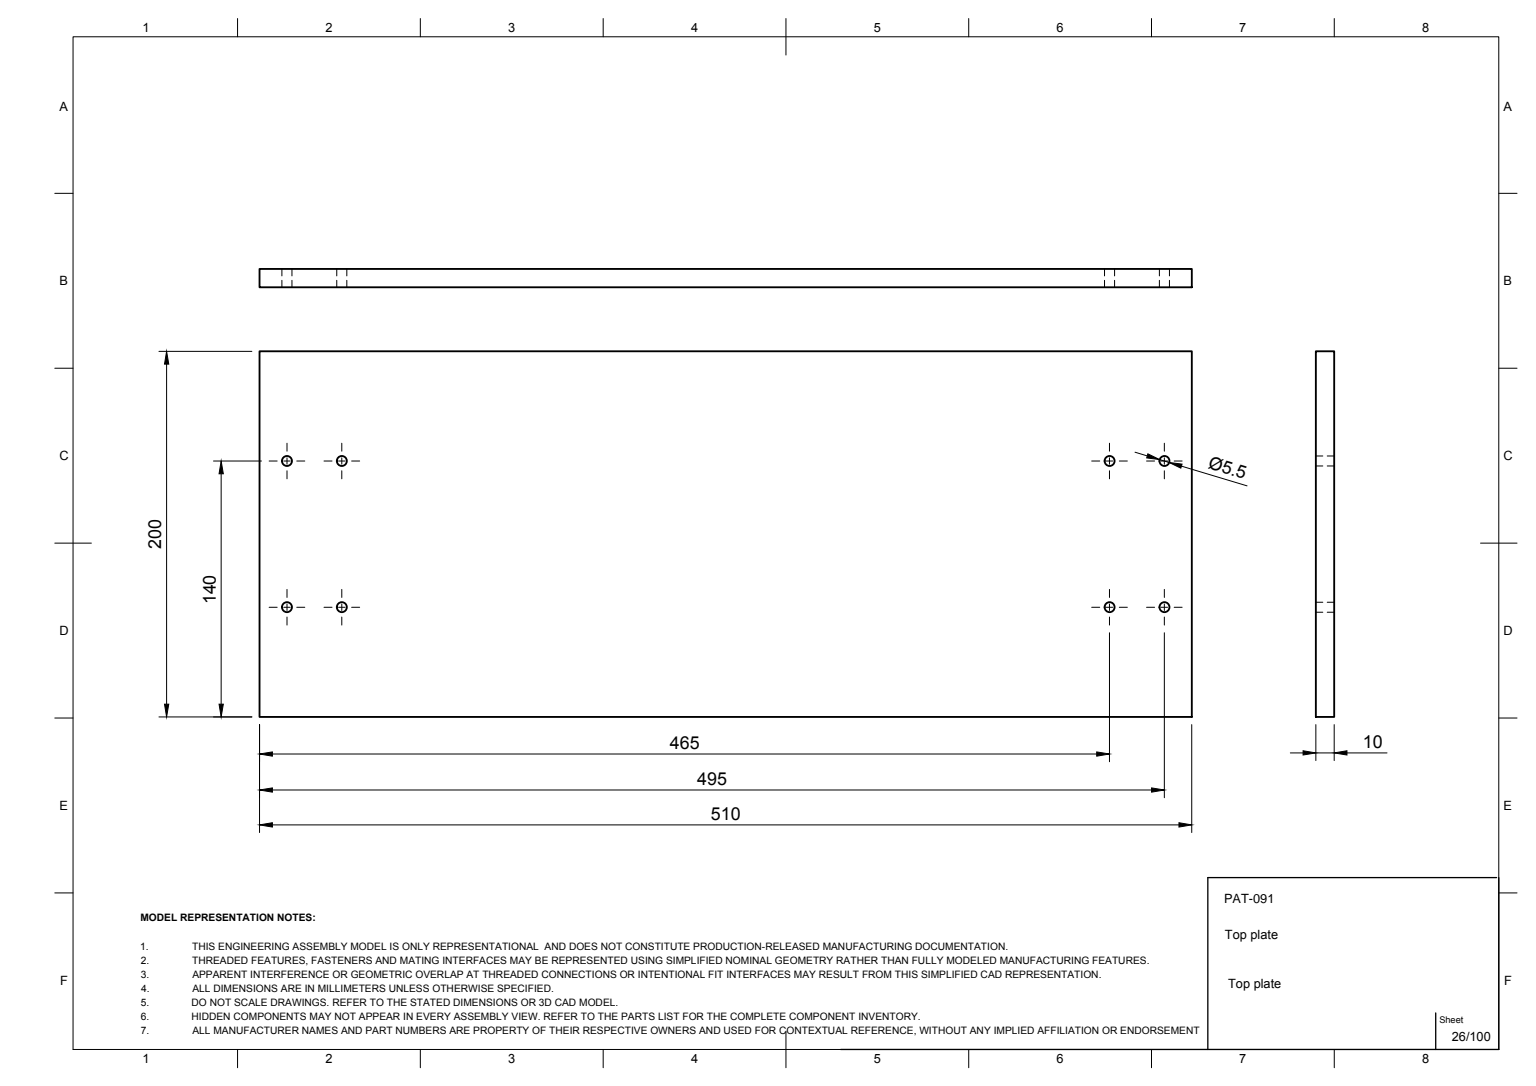
ISO-10303-21;
HEADER;
/* Generated by software containing ST-Developer
 * from STEP Tools, Inc. (www.steptools.com) 
 */

FILE_DESCRIPTION(
/* description */ ('PAT-091'),
/* implementation_level */ '2;1');

FILE_NAME(
/* name */ 'Top plate.step',
/* time_stamp */ '2026-10-27T15:34:44-07:00',
/* author */ (''),
/* organization */ (''),
/* preprocessor_version */ 'ST-DEVELOPER v20.2',
/* originating_system */ 'Autodesk Translation Framework v15.17.0.0',
/* authorisation */ '');

FILE_SCHEMA (('AUTOMOTIVE_DESIGN { 1 0 10303 214 3 1 1 }'));
ENDSEC;

DATA;
#10=MECHANICAL_DESIGN_GEOMETRIC_PRESENTATION_REPRESENTATION('',(#989),#25100);
#769=SHAPE_REPRESENTATION_RELATIONSHIP('SRR','None',#25531,#879);
#879=ADVANCED_BREP_SHAPE_REPRESENTATION('',(#1112),#25001);
#989=STYLED_ITEM('',(#26177),#1112);
#1112=MANIFOLD_SOLID_BREP('Body1',#13267);
#1334=FACE_BOUND('',#3171,.T.);
#1335=FACE_BOUND('',#3172,.T.);
#1336=FACE_BOUND('',#3173,.T.);
#1337=FACE_BOUND('',#3174,.T.);
#1338=FACE_BOUND('',#3175,.T.);
#1339=FACE_BOUND('',#3176,.T.);
#1340=FACE_BOUND('',#3177,.T.);
#1341=FACE_BOUND('',#3178,.T.);
#1342=FACE_BOUND('',#3180,.T.);
#1343=FACE_BOUND('',#3181,.T.);
#1344=FACE_BOUND('',#3182,.T.);
#1345=FACE_BOUND('',#3183,.T.);
#1346=FACE_BOUND('',#3184,.T.);
#1347=FACE_BOUND('',#3185,.T.);
#1348=FACE_BOUND('',#3186,.T.);
#1349=FACE_BOUND('',#3187,.T.);
#1719=PLANE('',#14944);
#1720=PLANE('',#14945);
#1721=PLANE('',#14946);
#1722=PLANE('',#14947);
#1723=PLANE('',#14948);
#1724=PLANE('',#14949);
#2221=FACE_OUTER_BOUND('',#3158,.T.);
#2222=FACE_OUTER_BOUND('',#3159,.T.);
#2223=FACE_OUTER_BOUND('',#3160,.T.);
#2224=FACE_OUTER_BOUND('',#3161,.T.);
#2225=FACE_OUTER_BOUND('',#3162,.T.);
#2226=FACE_OUTER_BOUND('',#3163,.T.);
#2227=FACE_OUTER_BOUND('',#3164,.T.);
#2228=FACE_OUTER_BOUND('',#3165,.T.);
#2229=FACE_OUTER_BOUND('',#3166,.T.);
#2230=FACE_OUTER_BOUND('',#3167,.T.);
#2231=FACE_OUTER_BOUND('',#3168,.T.);
#2232=FACE_OUTER_BOUND('',#3169,.T.);
#2233=FACE_OUTER_BOUND('',#3170,.T.);
#2234=FACE_OUTER_BOUND('',#3179,.T.);
#3158=EDGE_LOOP('',(#9644,#9645,#9646,#9647));
#3159=EDGE_LOOP('',(#9648,#9649,#9650,#9651));
#3160=EDGE_LOOP('',(#9652,#9653,#9654,#9655));
#3161=EDGE_LOOP('',(#9656,#9657,#9658,#9659));
#3162=EDGE_LOOP('',(#9660,#9661,#9662,#9663));
#3163=EDGE_LOOP('',(#9664,#9665,#9666,#9667));
#3164=EDGE_LOOP('',(#9668,#9669,#9670,#9671));
#3165=EDGE_LOOP('',(#9672,#9673,#9674,#9675));
#3166=EDGE_LOOP('',(#9676,#9677,#9678,#9679));
#3167=EDGE_LOOP('',(#9680,#9681,#9682,#9683));
#3168=EDGE_LOOP('',(#9684,#9685,#9686,#9687));
#3169=EDGE_LOOP('',(#9688,#9689,#9690,#9691));
#3170=EDGE_LOOP('',(#9692,#9693,#9694,#9695));
#3171=EDGE_LOOP('',(#9696));
#3172=EDGE_LOOP('',(#9697));
#3173=EDGE_LOOP('',(#9698));
#3174=EDGE_LOOP('',(#9699));
#3175=EDGE_LOOP('',(#9700));
#3176=EDGE_LOOP('',(#9701));
#3177=EDGE_LOOP('',(#9702));
#3178=EDGE_LOOP('',(#9703));
#3179=EDGE_LOOP('',(#9704,#9705,#9706,#9707));
#3180=EDGE_LOOP('',(#9708));
#3181=EDGE_LOOP('',(#9709));
#3182=EDGE_LOOP('',(#9710));
#3183=EDGE_LOOP('',(#9711));
#3184=EDGE_LOOP('',(#9712));
#3185=EDGE_LOOP('',(#9713));
#3186=EDGE_LOOP('',(#9714));
#3187=EDGE_LOOP('',(#9715));
#4305=LINE('',#21717,#5045);
#4306=LINE('',#21723,#5046);
#4307=LINE('',#21729,#5047);
#4308=LINE('',#21735,#5048);
#4309=LINE('',#21741,#5049);
#4310=LINE('',#21747,#5050);
#4311=LINE('',#21753,#5051);
#4312=LINE('',#21759,#5052);
#4313=LINE('',#21764,#5053);
#4314=LINE('',#21766,#5054);
#4315=LINE('',#21768,#5055);
#4316=LINE('',#21769,#5056);
#4317=LINE('',#21772,#5057);
#4318=LINE('',#21774,#5058);
#4319=LINE('',#21775,#5059);
#4320=LINE('',#21778,#5060);
#4321=LINE('',#21780,#5061);
#4322=LINE('',#21781,#5062);
#4323=LINE('',#21783,#5063);
#4324=LINE('',#21784,#5064);
#5045=VECTOR('',#17323,0.274999999999999);
#5046=VECTOR('',#17330,0.274999999999999);
#5047=VECTOR('',#17337,0.274999999999999);
#5048=VECTOR('',#17344,0.274999999999999);
#5049=VECTOR('',#17351,0.275);
#5050=VECTOR('',#17358,0.275);
#5051=VECTOR('',#17365,0.275);
#5052=VECTOR('',#17372,0.275);
#5053=VECTOR('',#17377,1.);
#5054=VECTOR('',#17378,1.);
#5055=VECTOR('',#17379,1.);
#5056=VECTOR('',#17380,1.);
#5057=VECTOR('',#17383,1.);
#5058=VECTOR('',#17384,1.);
#5059=VECTOR('',#17385,1.);
#5060=VECTOR('',#17388,1.);
#5061=VECTOR('',#17389,1.);
#5062=VECTOR('',#17390,1.);
#5063=VECTOR('',#17393,1.);
#5064=VECTOR('',#17394,1.);
#5759=CIRCLE('',#14921,0.274999999999999);
#5760=CIRCLE('',#14922,0.274999999999999);
#5761=CIRCLE('',#14924,0.274999999999999);
#5762=CIRCLE('',#14925,0.274999999999999);
#5763=CIRCLE('',#14927,0.274999999999999);
#5764=CIRCLE('',#14928,0.274999999999999);
#5765=CIRCLE('',#14930,0.274999999999999);
#5766=CIRCLE('',#14931,0.274999999999999);
#5767=CIRCLE('',#14933,0.275);
#5768=CIRCLE('',#14934,0.275);
#5769=CIRCLE('',#14936,0.275);
#5770=CIRCLE('',#14937,0.275);
#5771=CIRCLE('',#14939,0.275);
#5772=CIRCLE('',#14940,0.275);
#5773=CIRCLE('',#14942,0.275);
#5774=CIRCLE('',#14943,0.275);
#6606=VERTEX_POINT('',#21714);
#6607=VERTEX_POINT('',#21716);
#6608=VERTEX_POINT('',#21720);
#6609=VERTEX_POINT('',#21722);
#6610=VERTEX_POINT('',#21726);
#6611=VERTEX_POINT('',#21728);
#6612=VERTEX_POINT('',#21732);
#6613=VERTEX_POINT('',#21734);
#6614=VERTEX_POINT('',#21738);
#6615=VERTEX_POINT('',#21740);
#6616=VERTEX_POINT('',#21744);
#6617=VERTEX_POINT('',#21746);
#6618=VERTEX_POINT('',#21750);
#6619=VERTEX_POINT('',#21752);
#6620=VERTEX_POINT('',#21756);
#6621=VERTEX_POINT('',#21758);
#6622=VERTEX_POINT('',#21762);
#6623=VERTEX_POINT('',#21763);
#6624=VERTEX_POINT('',#21765);
#6625=VERTEX_POINT('',#21767);
#6626=VERTEX_POINT('',#21771);
#6627=VERTEX_POINT('',#21773);
#6628=VERTEX_POINT('',#21777);
#6629=VERTEX_POINT('',#21779);
#7757=EDGE_CURVE('',#6606,#6606,#5759,.T.);
#7758=EDGE_CURVE('',#6606,#6607,#4305,.T.);
#7759=EDGE_CURVE('',#6607,#6607,#5760,.T.);
#7760=EDGE_CURVE('',#6608,#6608,#5761,.T.);
#7761=EDGE_CURVE('',#6608,#6609,#4306,.T.);
#7762=EDGE_CURVE('',#6609,#6609,#5762,.T.);
#7763=EDGE_CURVE('',#6610,#6610,#5763,.T.);
#7764=EDGE_CURVE('',#6610,#6611,#4307,.T.);
#7765=EDGE_CURVE('',#6611,#6611,#5764,.T.);
#7766=EDGE_CURVE('',#6612,#6612,#5765,.T.);
#7767=EDGE_CURVE('',#6612,#6613,#4308,.T.);
#7768=EDGE_CURVE('',#6613,#6613,#5766,.T.);
#7769=EDGE_CURVE('',#6614,#6614,#5767,.T.);
#7770=EDGE_CURVE('',#6614,#6615,#4309,.T.);
#7771=EDGE_CURVE('',#6615,#6615,#5768,.T.);
#7772=EDGE_CURVE('',#6616,#6616,#5769,.T.);
#7773=EDGE_CURVE('',#6616,#6617,#4310,.T.);
#7774=EDGE_CURVE('',#6617,#6617,#5770,.T.);
#7775=EDGE_CURVE('',#6618,#6618,#5771,.T.);
#7776=EDGE_CURVE('',#6618,#6619,#4311,.T.);
#7777=EDGE_CURVE('',#6619,#6619,#5772,.T.);
#7778=EDGE_CURVE('',#6620,#6620,#5773,.T.);
#7779=EDGE_CURVE('',#6620,#6621,#4312,.T.);
#7780=EDGE_CURVE('',#6621,#6621,#5774,.T.);
#7781=EDGE_CURVE('',#6622,#6623,#4313,.T.);
#7782=EDGE_CURVE('',#6623,#6624,#4314,.T.);
#7783=EDGE_CURVE('',#6625,#6624,#4315,.T.);
#7784=EDGE_CURVE('',#6622,#6625,#4316,.T.);
#7785=EDGE_CURVE('',#6626,#6622,#4317,.T.);
#7786=EDGE_CURVE('',#6627,#6625,#4318,.T.);
#7787=EDGE_CURVE('',#6626,#6627,#4319,.T.);
#7788=EDGE_CURVE('',#6628,#6626,#4320,.T.);
#7789=EDGE_CURVE('',#6629,#6627,#4321,.T.);
#7790=EDGE_CURVE('',#6628,#6629,#4322,.T.);
#7791=EDGE_CURVE('',#6623,#6628,#4323,.T.);
#7792=EDGE_CURVE('',#6624,#6629,#4324,.T.);
#9644=ORIENTED_EDGE('',*,*,#7757,.F.);
#9645=ORIENTED_EDGE('',*,*,#7758,.T.);
#9646=ORIENTED_EDGE('',*,*,#7759,.F.);
#9647=ORIENTED_EDGE('',*,*,#7758,.F.);
#9648=ORIENTED_EDGE('',*,*,#7760,.F.);
#9649=ORIENTED_EDGE('',*,*,#7761,.T.);
#9650=ORIENTED_EDGE('',*,*,#7762,.F.);
#9651=ORIENTED_EDGE('',*,*,#7761,.F.);
#9652=ORIENTED_EDGE('',*,*,#7763,.F.);
#9653=ORIENTED_EDGE('',*,*,#7764,.T.);
#9654=ORIENTED_EDGE('',*,*,#7765,.F.);
#9655=ORIENTED_EDGE('',*,*,#7764,.F.);
#9656=ORIENTED_EDGE('',*,*,#7766,.F.);
#9657=ORIENTED_EDGE('',*,*,#7767,.T.);
#9658=ORIENTED_EDGE('',*,*,#7768,.F.);
#9659=ORIENTED_EDGE('',*,*,#7767,.F.);
#9660=ORIENTED_EDGE('',*,*,#7769,.F.);
#9661=ORIENTED_EDGE('',*,*,#7770,.T.);
#9662=ORIENTED_EDGE('',*,*,#7771,.F.);
#9663=ORIENTED_EDGE('',*,*,#7770,.F.);
#9664=ORIENTED_EDGE('',*,*,#7772,.F.);
#9665=ORIENTED_EDGE('',*,*,#7773,.T.);
#9666=ORIENTED_EDGE('',*,*,#7774,.F.);
#9667=ORIENTED_EDGE('',*,*,#7773,.F.);
#9668=ORIENTED_EDGE('',*,*,#7775,.F.);
#9669=ORIENTED_EDGE('',*,*,#7776,.T.);
#9670=ORIENTED_EDGE('',*,*,#7777,.F.);
#9671=ORIENTED_EDGE('',*,*,#7776,.F.);
#9672=ORIENTED_EDGE('',*,*,#7778,.F.);
#9673=ORIENTED_EDGE('',*,*,#7779,.T.);
#9674=ORIENTED_EDGE('',*,*,#7780,.F.);
#9675=ORIENTED_EDGE('',*,*,#7779,.F.);
#9676=ORIENTED_EDGE('',*,*,#7781,.T.);
#9677=ORIENTED_EDGE('',*,*,#7782,.T.);
#9678=ORIENTED_EDGE('',*,*,#7783,.F.);
#9679=ORIENTED_EDGE('',*,*,#7784,.F.);
#9680=ORIENTED_EDGE('',*,*,#7785,.T.);
#9681=ORIENTED_EDGE('',*,*,#7784,.T.);
#9682=ORIENTED_EDGE('',*,*,#7786,.F.);
#9683=ORIENTED_EDGE('',*,*,#7787,.F.);
#9684=ORIENTED_EDGE('',*,*,#7788,.T.);
#9685=ORIENTED_EDGE('',*,*,#7787,.T.);
#9686=ORIENTED_EDGE('',*,*,#7789,.F.);
#9687=ORIENTED_EDGE('',*,*,#7790,.F.);
#9688=ORIENTED_EDGE('',*,*,#7791,.T.);
#9689=ORIENTED_EDGE('',*,*,#7790,.T.);
#9690=ORIENTED_EDGE('',*,*,#7792,.F.);
#9691=ORIENTED_EDGE('',*,*,#7782,.F.);
#9692=ORIENTED_EDGE('',*,*,#7792,.T.);
#9693=ORIENTED_EDGE('',*,*,#7789,.T.);
#9694=ORIENTED_EDGE('',*,*,#7786,.T.);
#9695=ORIENTED_EDGE('',*,*,#7783,.T.);
#9696=ORIENTED_EDGE('',*,*,#7780,.T.);
#9697=ORIENTED_EDGE('',*,*,#7777,.T.);
#9698=ORIENTED_EDGE('',*,*,#7774,.T.);
#9699=ORIENTED_EDGE('',*,*,#7771,.T.);
#9700=ORIENTED_EDGE('',*,*,#7768,.T.);
#9701=ORIENTED_EDGE('',*,*,#7765,.T.);
#9702=ORIENTED_EDGE('',*,*,#7762,.T.);
#9703=ORIENTED_EDGE('',*,*,#7759,.T.);
#9704=ORIENTED_EDGE('',*,*,#7791,.F.);
#9705=ORIENTED_EDGE('',*,*,#7781,.F.);
#9706=ORIENTED_EDGE('',*,*,#7785,.F.);
#9707=ORIENTED_EDGE('',*,*,#7788,.F.);
#9708=ORIENTED_EDGE('',*,*,#7778,.T.);
#9709=ORIENTED_EDGE('',*,*,#7775,.T.);
#9710=ORIENTED_EDGE('',*,*,#7772,.T.);
#9711=ORIENTED_EDGE('',*,*,#7769,.T.);
#9712=ORIENTED_EDGE('',*,*,#7766,.T.);
#9713=ORIENTED_EDGE('',*,*,#7763,.T.);
#9714=ORIENTED_EDGE('',*,*,#7760,.T.);
#9715=ORIENTED_EDGE('',*,*,#7757,.T.);
#12150=CYLINDRICAL_SURFACE('',#14920,0.274999999999999);
#12151=CYLINDRICAL_SURFACE('',#14923,0.274999999999999);
#12152=CYLINDRICAL_SURFACE('',#14926,0.274999999999999);
#12153=CYLINDRICAL_SURFACE('',#14929,0.274999999999999);
#12154=CYLINDRICAL_SURFACE('',#14932,0.275);
#12155=CYLINDRICAL_SURFACE('',#14935,0.275);
#12156=CYLINDRICAL_SURFACE('',#14938,0.275);
#12157=CYLINDRICAL_SURFACE('',#14941,0.275);
#12588=ADVANCED_FACE('',(#2221),#12150,.F.);
#12589=ADVANCED_FACE('',(#2222),#12151,.F.);
#12590=ADVANCED_FACE('',(#2223),#12152,.F.);
#12591=ADVANCED_FACE('',(#2224),#12153,.F.);
#12592=ADVANCED_FACE('',(#2225),#12154,.F.);
#12593=ADVANCED_FACE('',(#2226),#12155,.F.);
#12594=ADVANCED_FACE('',(#2227),#12156,.F.);
#12595=ADVANCED_FACE('',(#2228),#12157,.F.);
#12596=ADVANCED_FACE('',(#2229),#1719,.T.);
#12597=ADVANCED_FACE('',(#2230),#1720,.T.);
#12598=ADVANCED_FACE('',(#2231),#1721,.T.);
#12599=ADVANCED_FACE('',(#2232),#1722,.T.);
#12600=ADVANCED_FACE('',(#2233,#1334,#1335,#1336,#1337,#1338,#1339,#1340,
#1341),#1723,.T.);
#12601=ADVANCED_FACE('',(#2234,#1342,#1343,#1344,#1345,#1346,#1347,#1348,
#1349),#1724,.F.);
#13267=CLOSED_SHELL('',(#12588,#12589,#12590,#12591,#12592,#12593,#12594,
#12595,#12596,#12597,#12598,#12599,#12600,#12601));
#14919=AXIS2_PLACEMENT_3D('',#21712,#17317,#17318);
#14920=AXIS2_PLACEMENT_3D('',#21713,#17319,#17320);
#14921=AXIS2_PLACEMENT_3D('',#21715,#17321,#17322);
#14922=AXIS2_PLACEMENT_3D('',#21718,#17324,#17325);
#14923=AXIS2_PLACEMENT_3D('',#21719,#17326,#17327);
#14924=AXIS2_PLACEMENT_3D('',#21721,#17328,#17329);
#14925=AXIS2_PLACEMENT_3D('',#21724,#17331,#17332);
#14926=AXIS2_PLACEMENT_3D('',#21725,#17333,#17334);
#14927=AXIS2_PLACEMENT_3D('',#21727,#17335,#17336);
#14928=AXIS2_PLACEMENT_3D('',#21730,#17338,#17339);
#14929=AXIS2_PLACEMENT_3D('',#21731,#17340,#17341);
#14930=AXIS2_PLACEMENT_3D('',#21733,#17342,#17343);
#14931=AXIS2_PLACEMENT_3D('',#21736,#17345,#17346);
#14932=AXIS2_PLACEMENT_3D('',#21737,#17347,#17348);
#14933=AXIS2_PLACEMENT_3D('',#21739,#17349,#17350);
#14934=AXIS2_PLACEMENT_3D('',#21742,#17352,#17353);
#14935=AXIS2_PLACEMENT_3D('',#21743,#17354,#17355);
#14936=AXIS2_PLACEMENT_3D('',#21745,#17356,#17357);
#14937=AXIS2_PLACEMENT_3D('',#21748,#17359,#17360);
#14938=AXIS2_PLACEMENT_3D('',#21749,#17361,#17362);
#14939=AXIS2_PLACEMENT_3D('',#21751,#17363,#17364);
#14940=AXIS2_PLACEMENT_3D('',#21754,#17366,#17367);
#14941=AXIS2_PLACEMENT_3D('',#21755,#17368,#17369);
#14942=AXIS2_PLACEMENT_3D('',#21757,#17370,#17371);
#14943=AXIS2_PLACEMENT_3D('',#21760,#17373,#17374);
#14944=AXIS2_PLACEMENT_3D('',#21761,#17375,#17376);
#14945=AXIS2_PLACEMENT_3D('',#21770,#17381,#17382);
#14946=AXIS2_PLACEMENT_3D('',#21776,#17386,#17387);
#14947=AXIS2_PLACEMENT_3D('',#21782,#17391,#17392);
#14948=AXIS2_PLACEMENT_3D('',#21785,#17395,#17396);
#14949=AXIS2_PLACEMENT_3D('',#21786,#17397,#17398);
#17317=DIRECTION('axis',(0.,0.,1.));
#17318=DIRECTION('refdir',(1.,0.,0.));
#17319=DIRECTION('center_axis',(0.,0.,1.));
#17320=DIRECTION('ref_axis',(1.,0.,0.));
#17321=DIRECTION('center_axis',(0.,0.,1.));
#17322=DIRECTION('ref_axis',(1.,0.,0.));
#17323=DIRECTION('',(0.,0.,1.));
#17324=DIRECTION('center_axis',(0.,0.,-1.));
#17325=DIRECTION('ref_axis',(1.,0.,0.));
#17326=DIRECTION('center_axis',(0.,0.,1.));
#17327=DIRECTION('ref_axis',(1.,0.,0.));
#17328=DIRECTION('center_axis',(0.,0.,1.));
#17329=DIRECTION('ref_axis',(1.,0.,0.));
#17330=DIRECTION('',(0.,0.,1.));
#17331=DIRECTION('center_axis',(0.,0.,-1.));
#17332=DIRECTION('ref_axis',(1.,0.,0.));
#17333=DIRECTION('center_axis',(0.,0.,1.));
#17334=DIRECTION('ref_axis',(1.,0.,0.));
#17335=DIRECTION('center_axis',(0.,0.,1.));
#17336=DIRECTION('ref_axis',(1.,0.,0.));
#17337=DIRECTION('',(0.,0.,1.));
#17338=DIRECTION('center_axis',(0.,0.,-1.));
#17339=DIRECTION('ref_axis',(1.,0.,0.));
#17340=DIRECTION('center_axis',(0.,0.,1.));
#17341=DIRECTION('ref_axis',(1.,0.,0.));
#17342=DIRECTION('center_axis',(0.,0.,1.));
#17343=DIRECTION('ref_axis',(1.,0.,0.));
#17344=DIRECTION('',(0.,0.,1.));
#17345=DIRECTION('center_axis',(0.,0.,-1.));
#17346=DIRECTION('ref_axis',(1.,0.,0.));
#17347=DIRECTION('center_axis',(0.,0.,1.));
#17348=DIRECTION('ref_axis',(1.,0.,0.));
#17349=DIRECTION('center_axis',(0.,0.,1.));
#17350=DIRECTION('ref_axis',(1.,0.,0.));
#17351=DIRECTION('',(0.,0.,1.));
#17352=DIRECTION('center_axis',(0.,0.,-1.));
#17353=DIRECTION('ref_axis',(1.,0.,0.));
#17354=DIRECTION('center_axis',(0.,0.,1.));
#17355=DIRECTION('ref_axis',(1.,0.,0.));
#17356=DIRECTION('center_axis',(0.,0.,1.));
#17357=DIRECTION('ref_axis',(1.,0.,0.));
#17358=DIRECTION('',(0.,0.,1.));
#17359=DIRECTION('center_axis',(0.,0.,-1.));
#17360=DIRECTION('ref_axis',(1.,0.,0.));
#17361=DIRECTION('center_axis',(0.,0.,1.));
#17362=DIRECTION('ref_axis',(1.,0.,0.));
#17363=DIRECTION('center_axis',(0.,0.,1.));
#17364=DIRECTION('ref_axis',(1.,0.,0.));
#17365=DIRECTION('',(0.,0.,1.));
#17366=DIRECTION('center_axis',(0.,0.,-1.));
#17367=DIRECTION('ref_axis',(1.,0.,0.));
#17368=DIRECTION('center_axis',(0.,0.,1.));
#17369=DIRECTION('ref_axis',(1.,0.,0.));
#17370=DIRECTION('center_axis',(0.,0.,1.));
#17371=DIRECTION('ref_axis',(1.,0.,0.));
#17372=DIRECTION('',(0.,0.,1.));
#17373=DIRECTION('center_axis',(0.,0.,-1.));
#17374=DIRECTION('ref_axis',(1.,0.,0.));
#17375=DIRECTION('center_axis',(0.,1.,0.));
#17376=DIRECTION('ref_axis',(-1.,0.,0.));
#17377=DIRECTION('',(-1.,0.,0.));
#17378=DIRECTION('',(0.,0.,1.));
#17379=DIRECTION('',(-1.,0.,0.));
#17380=DIRECTION('',(0.,0.,1.));
#17381=DIRECTION('center_axis',(1.,0.,0.));
#17382=DIRECTION('ref_axis',(0.,1.,0.));
#17383=DIRECTION('',(0.,1.,0.));
#17384=DIRECTION('',(0.,1.,0.));
#17385=DIRECTION('',(0.,0.,1.));
#17386=DIRECTION('center_axis',(0.,-1.,0.));
#17387=DIRECTION('ref_axis',(1.,0.,0.));
#17388=DIRECTION('',(1.,0.,0.));
#17389=DIRECTION('',(1.,0.,0.));
#17390=DIRECTION('',(0.,0.,1.));
#17391=DIRECTION('center_axis',(-1.,0.,0.));
#17392=DIRECTION('ref_axis',(0.,-1.,0.));
#17393=DIRECTION('',(0.,-1.,0.));
#17394=DIRECTION('',(0.,-1.,0.));
#17395=DIRECTION('center_axis',(0.,0.,1.));
#17396=DIRECTION('ref_axis',(1.,0.,0.));
#17397=DIRECTION('center_axis',(0.,0.,1.));
#17398=DIRECTION('ref_axis',(1.,0.,0.));
#21712=CARTESIAN_POINT('',(0.,0.,0.));
#21713=CARTESIAN_POINT('Origin',(46.5,-4.,17.9));
#21714=CARTESIAN_POINT('',(46.225,-4.,18.));
#21715=CARTESIAN_POINT('Origin',(46.5,-4.,18.));
#21716=CARTESIAN_POINT('',(46.225,-4.,19.));
#21717=CARTESIAN_POINT('',(46.225,-4.,17.9));
#21718=CARTESIAN_POINT('Origin',(46.5,-4.,19.));
#21719=CARTESIAN_POINT('Origin',(43.5,4.,17.9));
#21720=CARTESIAN_POINT('',(43.225,4.,18.));
#21721=CARTESIAN_POINT('Origin',(43.5,4.,18.));
#21722=CARTESIAN_POINT('',(43.225,4.,19.));
#21723=CARTESIAN_POINT('',(43.225,4.,17.9));
#21724=CARTESIAN_POINT('Origin',(43.5,4.,19.));
#21725=CARTESIAN_POINT('Origin',(43.5,-4.,17.9));
#21726=CARTESIAN_POINT('',(43.225,-4.,18.));
#21727=CARTESIAN_POINT('Origin',(43.5,-4.,18.));
#21728=CARTESIAN_POINT('',(43.225,-4.,19.));
#21729=CARTESIAN_POINT('',(43.225,-4.,17.9));
#21730=CARTESIAN_POINT('Origin',(43.5,-4.,19.));
#21731=CARTESIAN_POINT('Origin',(46.5,4.,17.9));
#21732=CARTESIAN_POINT('',(46.225,4.,18.));
#21733=CARTESIAN_POINT('Origin',(46.5,4.,18.));
#21734=CARTESIAN_POINT('',(46.225,4.,19.));
#21735=CARTESIAN_POINT('',(46.225,4.,17.9));
#21736=CARTESIAN_POINT('Origin',(46.5,4.,19.));
#21737=CARTESIAN_POINT('Origin',(1.5,-4.,17.9));
#21738=CARTESIAN_POINT('',(1.225,-4.,18.));
#21739=CARTESIAN_POINT('Origin',(1.5,-4.,18.));
#21740=CARTESIAN_POINT('',(1.225,-4.,19.));
#21741=CARTESIAN_POINT('',(1.225,-4.,17.9));
#21742=CARTESIAN_POINT('Origin',(1.5,-4.,19.));
#21743=CARTESIAN_POINT('Origin',(-1.5,4.,17.9));
#21744=CARTESIAN_POINT('',(-1.775,4.,18.));
#21745=CARTESIAN_POINT('Origin',(-1.5,4.,18.));
#21746=CARTESIAN_POINT('',(-1.775,4.,19.));
#21747=CARTESIAN_POINT('',(-1.775,4.,17.9));
#21748=CARTESIAN_POINT('Origin',(-1.5,4.,19.));
#21749=CARTESIAN_POINT('Origin',(-1.5,-4.,17.9));
#21750=CARTESIAN_POINT('',(-1.775,-4.,18.));
#21751=CARTESIAN_POINT('Origin',(-1.5,-4.,18.));
#21752=CARTESIAN_POINT('',(-1.775,-4.,19.));
#21753=CARTESIAN_POINT('',(-1.775,-4.,17.9));
#21754=CARTESIAN_POINT('Origin',(-1.5,-4.,19.));
#21755=CARTESIAN_POINT('Origin',(1.5,4.,17.9));
#21756=CARTESIAN_POINT('',(1.225,4.,18.));
#21757=CARTESIAN_POINT('Origin',(1.5,4.,18.));
#21758=CARTESIAN_POINT('',(1.225,4.,19.));
#21759=CARTESIAN_POINT('',(1.225,4.,17.9));
#21760=CARTESIAN_POINT('Origin',(1.5,4.,19.));
#21761=CARTESIAN_POINT('Origin',(48.,10.,18.));
#21762=CARTESIAN_POINT('',(48.,10.,18.));
#21763=CARTESIAN_POINT('',(-3.,10.,18.));
#21764=CARTESIAN_POINT('',(48.,10.,18.));
#21765=CARTESIAN_POINT('',(-3.,10.,19.));
#21766=CARTESIAN_POINT('',(-3.,10.,18.));
#21767=CARTESIAN_POINT('',(48.,10.,19.));
#21768=CARTESIAN_POINT('',(48.,10.,19.));
#21769=CARTESIAN_POINT('',(48.,10.,18.));
#21770=CARTESIAN_POINT('Origin',(48.,-10.,18.));
#21771=CARTESIAN_POINT('',(48.,-10.,18.));
#21772=CARTESIAN_POINT('',(48.,-10.,18.));
#21773=CARTESIAN_POINT('',(48.,-10.,19.));
#21774=CARTESIAN_POINT('',(48.,-10.,19.));
#21775=CARTESIAN_POINT('',(48.,-10.,18.));
#21776=CARTESIAN_POINT('Origin',(-3.,-10.,18.));
#21777=CARTESIAN_POINT('',(-3.,-10.,18.));
#21778=CARTESIAN_POINT('',(-3.,-10.,18.));
#21779=CARTESIAN_POINT('',(-3.,-10.,19.));
#21780=CARTESIAN_POINT('',(-3.,-10.,19.));
#21781=CARTESIAN_POINT('',(-3.,-10.,18.));
#21782=CARTESIAN_POINT('Origin',(-3.,10.,18.));
#21783=CARTESIAN_POINT('',(-3.,10.,18.));
#21784=CARTESIAN_POINT('',(-3.,10.,19.));
#21785=CARTESIAN_POINT('Origin',(22.5,0.,19.));
#21786=CARTESIAN_POINT('Origin',(22.5,0.,18.));
#24880=UNCERTAINTY_MEASURE_WITH_UNIT(LENGTH_MEASURE(0.001),#25101,
'DISTANCE_ACCURACY_VALUE',
'Maximum model space distance between geometric entities at asserted c
onnectivities');
#24979=UNCERTAINTY_MEASURE_WITH_UNIT(LENGTH_MEASURE(0.001),#25101,
'DISTANCE_ACCURACY_VALUE',
'Maximum model space distance between geometric entities at asserted c
onnectivities');
#25001=(
GEOMETRIC_REPRESENTATION_CONTEXT(3)
GLOBAL_UNCERTAINTY_ASSIGNED_CONTEXT((#24880))
GLOBAL_UNIT_ASSIGNED_CONTEXT((#25101,#25103,#25104))
REPRESENTATION_CONTEXT('','3D')
);
#25100=(
GEOMETRIC_REPRESENTATION_CONTEXT(3)
GLOBAL_UNCERTAINTY_ASSIGNED_CONTEXT((#24979))
GLOBAL_UNIT_ASSIGNED_CONTEXT((#25101,#25103,#25104))
REPRESENTATION_CONTEXT('','3D')
);
#25101=(
LENGTH_UNIT()
NAMED_UNIT(*)
SI_UNIT(.CENTI.,.METRE.)
);
#25103=(
NAMED_UNIT(*)
PLANE_ANGLE_UNIT()
SI_UNIT($,.RADIAN.)
);
#25104=(
NAMED_UNIT(*)
SI_UNIT($,.STERADIAN.)
SOLID_ANGLE_UNIT()
);
#25126=SHAPE_DEFINITION_REPRESENTATION(#25246,#25531);
#25246=PRODUCT_DEFINITION_SHAPE('',$,#25652);
#25531=SHAPE_REPRESENTATION('',(#14919),#25001);
#25630=PRODUCT_DEFINITION_CONTEXT('part definition',#25992,'design');
#25652=PRODUCT_DEFINITION('Top plate','Top plate',#25772,#25630);
#25772=PRODUCT_DEFINITION_FORMATION('',$,#26015);
#25992=APPLICATION_CONTEXT(
'Core Data for Automotive Mechanical Design Process');
#25993=PRODUCT_CONTEXT('part definition',#25992,'mechanical');
#26015=PRODUCT('Top plate','Top plate','Top plate',(#25993));
#26171=COLOUR_RGB('Light Blue',0.38,0.62,0.78);
#26172=FILL_AREA_STYLE_COLOUR('',#26171);
#26173=FILL_AREA_STYLE('',(#26172));
#26174=SURFACE_STYLE_FILL_AREA(#26173);
#26175=SURFACE_SIDE_STYLE('',(#26174));
#26176=SURFACE_STYLE_USAGE(.BOTH.,#26175);
#26177=PRESENTATION_STYLE_ASSIGNMENT((#26176));
ENDSEC;
END-ISO-10303-21;
